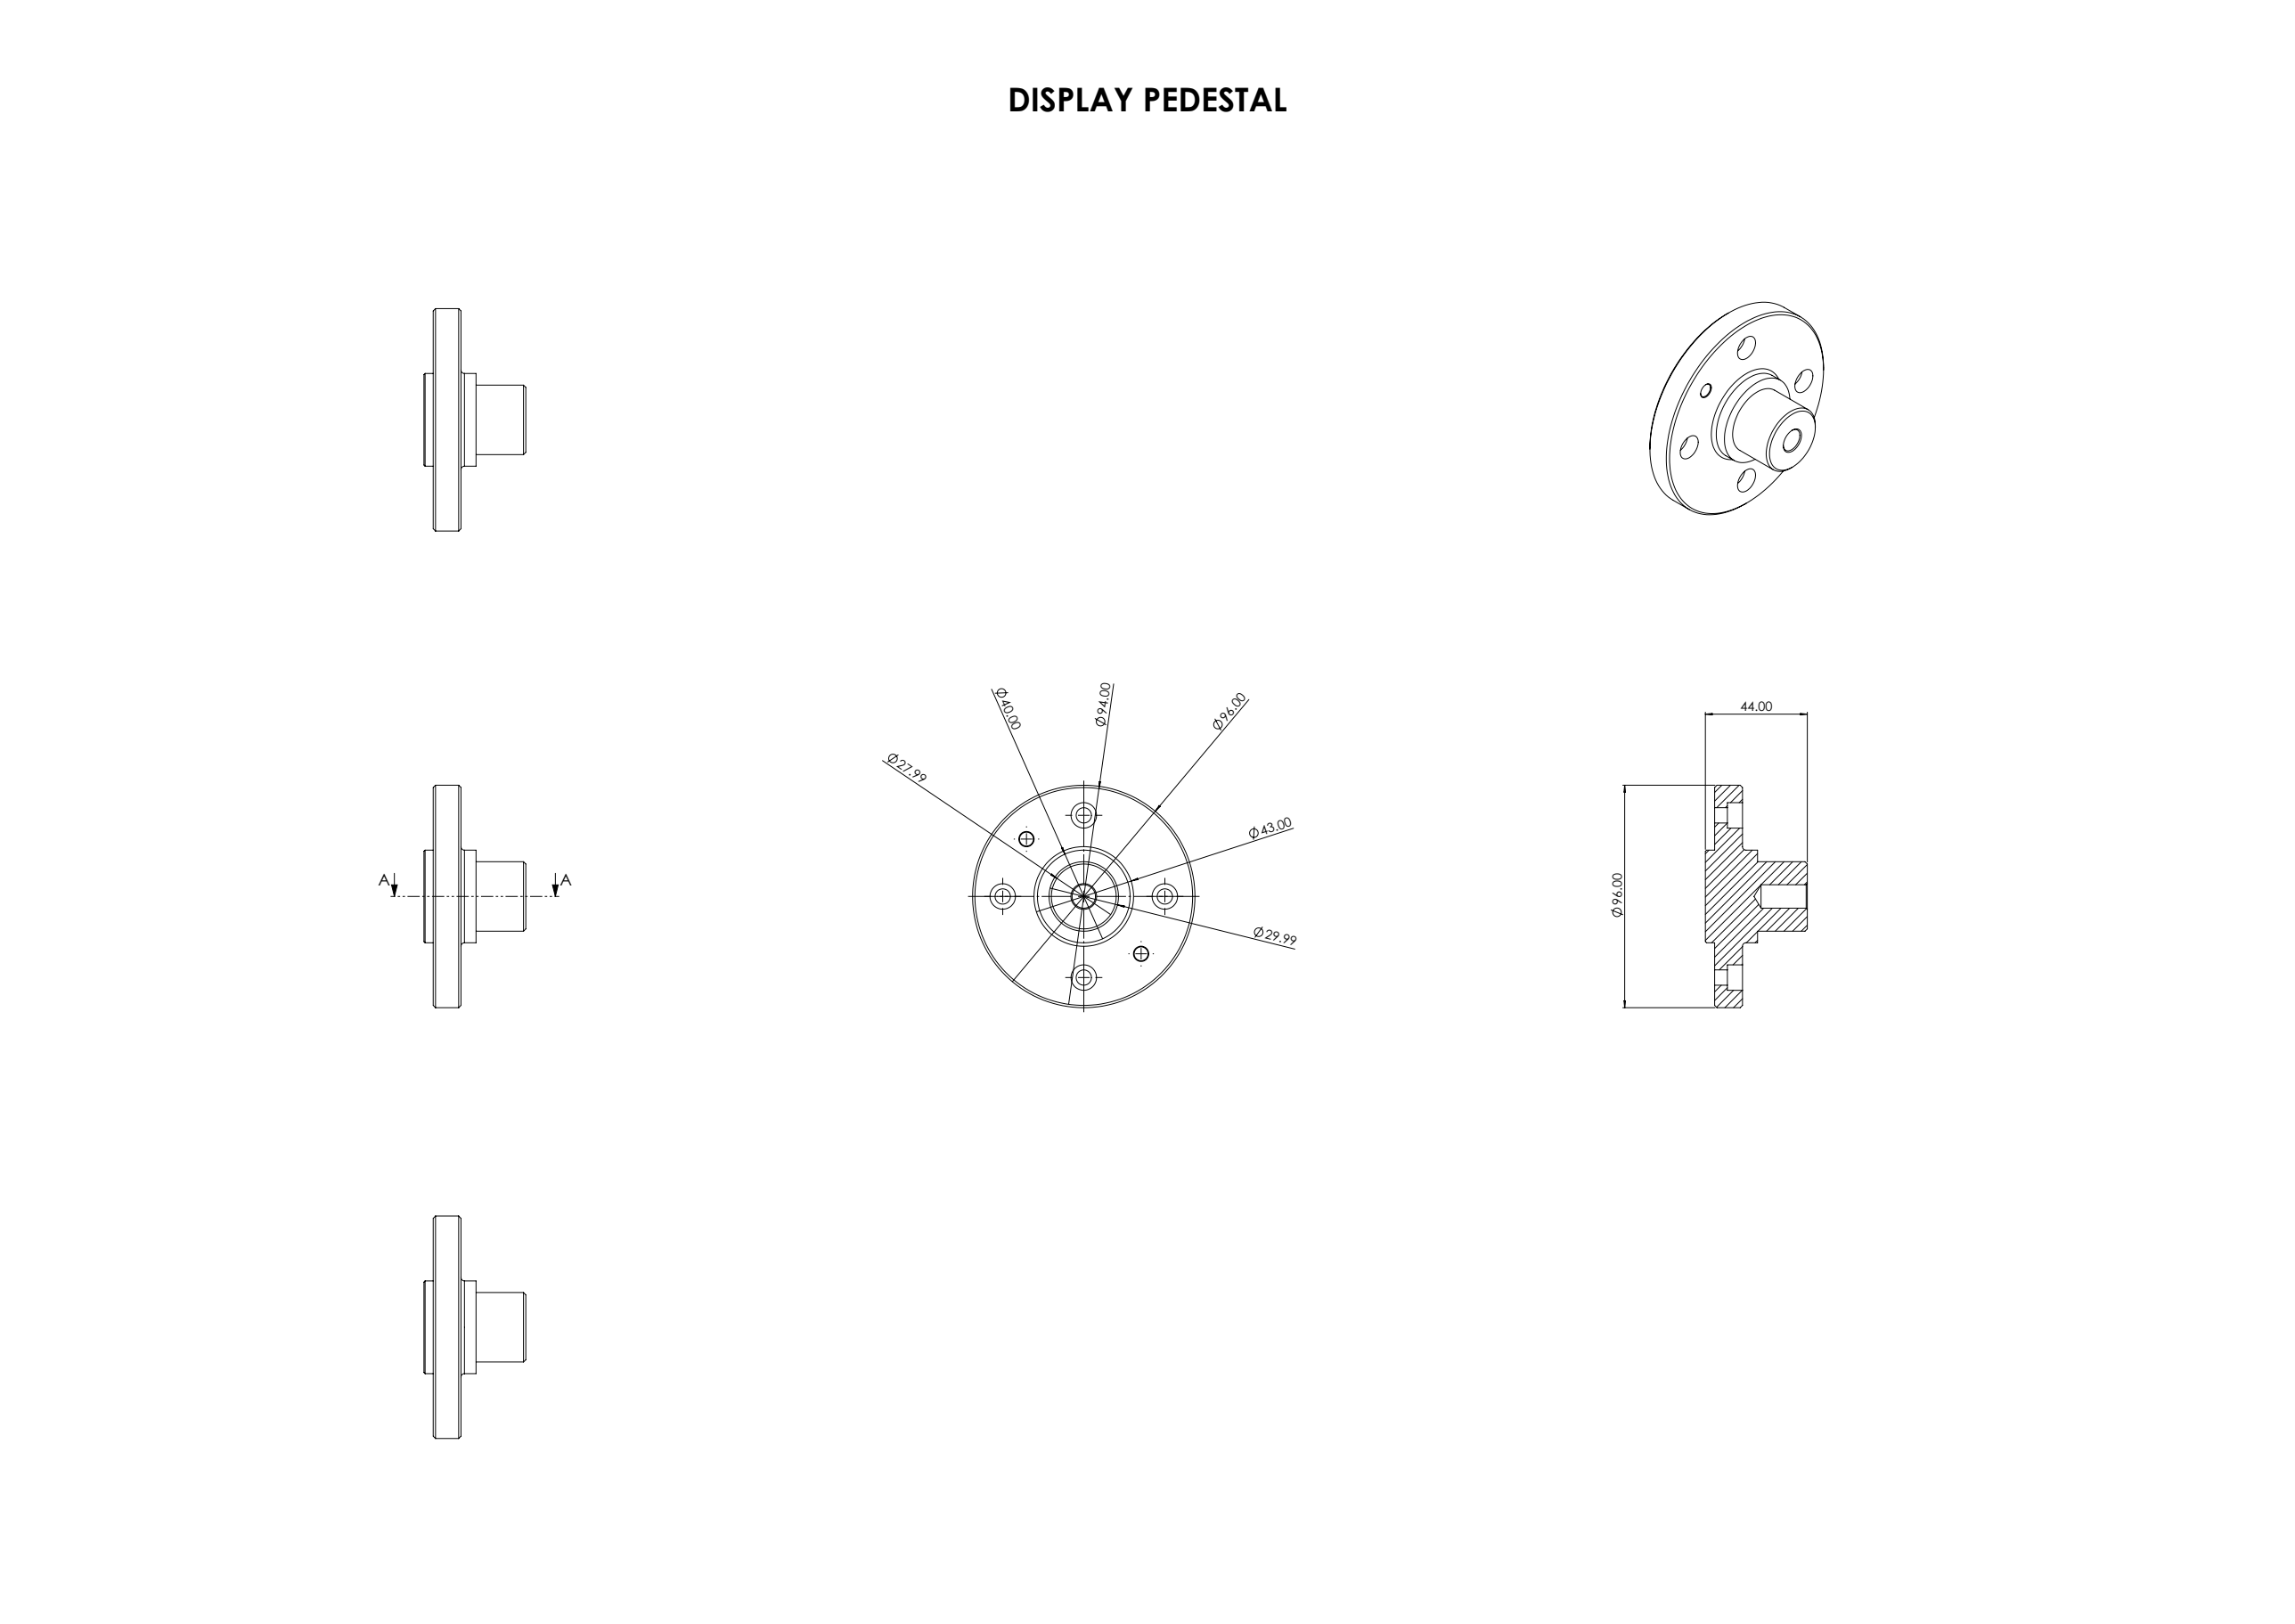
ISO-10303-21;
HEADER;
/* Generated by software containing ST-Developer
 * from STEP Tools, Inc. (www.steptools.com) 
 */

FILE_DESCRIPTION(
/* description */ (''),
/* implementation_level */ '2;1');

FILE_NAME(
/* name */ '03_Display_Pedestal.step',
/* time_stamp */ '2026-10-11T08:27:52-07:00',
/* author */ (''),
/* organization */ (''),
/* preprocessor_version */ 'ST-DEVELOPER v20.2',
/* originating_system */ 'Autodesk Translation Framework v15.15.0.0',
/* authorisation */ '');

FILE_SCHEMA (('AUTOMOTIVE_DESIGN { 1 0 10303 214 3 1 1 }'));
ENDSEC;

DATA;
#10=MECHANICAL_DESIGN_GEOMETRIC_PRESENTATION_REPRESENTATION('',(#921),#94301);
#893=SHAPE_REPRESENTATION_RELATIONSHIP('SRR','None',#94373,#907);
#907=ADVANCED_BREP_SHAPE_REPRESENTATION('',(#935),#94289);
#921=STYLED_ITEM('',(#94574),#935);
#935=MANIFOLD_SOLID_BREP('Body1',#51020);
#954=TOROIDAL_SURFACE('',#54190,21.5,1.5);
#969=FACE_BOUND('',#17694,.T.);
#970=FACE_BOUND('',#17695,.T.);
#971=FACE_BOUND('',#17696,.T.);
#972=FACE_BOUND('',#17697,.T.);
#973=FACE_BOUND('',#17698,.T.);
#974=FACE_BOUND('',#17699,.T.);
#975=FACE_BOUND('',#17700,.T.);
#976=FACE_BOUND('',#17710,.T.);
#977=FACE_BOUND('',#17713,.T.);
#978=FACE_BOUND('',#17716,.T.);
#979=FACE_BOUND('',#17719,.T.);
#980=FACE_BOUND('',#17729,.T.);
#981=FACE_BOUND('',#17730,.T.);
#982=FACE_BOUND('',#17731,.T.);
#983=FACE_BOUND('',#17732,.T.);
#984=FACE_BOUND('',#17733,.T.);
#985=FACE_BOUND('',#17734,.T.);
#986=FACE_BOUND('',#17735,.T.);
#987=FACE_BOUND('',#17740,.T.);
#988=FACE_BOUND('',#17744,.T.);
#1125=CYLINDRICAL_SURFACE('',#54154,3.);
#1126=CYLINDRICAL_SURFACE('',#54158,3.);
#1127=CYLINDRICAL_SURFACE('',#54160,3.3);
#1128=CYLINDRICAL_SURFACE('',#54163,3.3);
#1129=CYLINDRICAL_SURFACE('',#54166,3.3);
#1130=CYLINDRICAL_SURFACE('',#54169,3.3);
#1131=CYLINDRICAL_SURFACE('',#54172,5.5);
#1132=CYLINDRICAL_SURFACE('',#54175,5.5);
#1133=CYLINDRICAL_SURFACE('',#54178,5.5);
#1134=CYLINDRICAL_SURFACE('',#54181,5.5);
#1135=CYLINDRICAL_SURFACE('',#54186,5.05);
#1136=CYLINDRICAL_SURFACE('',#54194,20.);
#1137=CYLINDRICAL_SURFACE('',#54200,20.);
#1138=CYLINDRICAL_SURFACE('',#54206,48.);
#1139=CYLINDRICAL_SURFACE('',#54211,14.995);
#5334=LINE('',#80394,#9862);
#5335=LINE('',#80414,#9863);
#5336=LINE('',#80417,#9864);
#5337=LINE('',#80422,#9865);
#5338=LINE('',#80427,#9866);
#5339=LINE('',#80433,#9867);
#5340=LINE('',#80439,#9868);
#5341=LINE('',#80445,#9869);
#5342=LINE('',#80450,#9870);
#5343=LINE('',#80455,#9871);
#5344=LINE('',#80460,#9872);
#5345=LINE('',#80465,#9873);
#5346=LINE('',#80470,#9874);
#5347=LINE('',#80474,#9875);
#5348=LINE('',#80478,#9876);
#5349=LINE('',#80489,#9877);
#5350=LINE('',#80496,#9878);
#5351=LINE('',#80500,#9879);
#5352=LINE('',#80507,#9880);
#5353=LINE('',#80511,#9881);
#5354=LINE('',#80513,#9882);
#5355=LINE('',#80520,#9883);
#5356=LINE('',#80524,#9884);
#9862=VECTOR('',#64458,3.15);
#9863=VECTOR('',#64481,3.);
#9864=VECTOR('',#64484,3.15);
#9865=VECTOR('',#64491,3.);
#9866=VECTOR('',#64496,3.3);
#9867=VECTOR('',#64503,3.3);
#9868=VECTOR('',#64510,3.3);
#9869=VECTOR('',#64517,3.3);
#9870=VECTOR('',#64524,5.5);
#9871=VECTOR('',#64531,5.5);
#9872=VECTOR('',#64538,5.5);
#9873=VECTOR('',#64545,5.5);
#9874=VECTOR('',#64550,2.525);
#9875=VECTOR('',#64555,5.05);
#9876=VECTOR('',#64560,5.35);
#9877=VECTOR('',#64575,20.);
#9878=VECTOR('',#64584,19.75);
#9879=VECTOR('',#64589,20.);
#9880=VECTOR('',#64598,47.5);
#9881=VECTOR('',#64603,48.);
#9882=VECTOR('',#64606,47.5);
#9883=VECTOR('',#64615,14.995);
#9884=VECTOR('',#64620,14.495);
#12726=PLANE('',#54146);
#12727=PLANE('',#54174);
#12728=PLANE('',#54177);
#12729=PLANE('',#54180);
#12730=PLANE('',#54183);
#12731=PLANE('',#54196);
#12732=PLANE('',#54202);
#12733=PLANE('',#54209);
#12734=PLANE('',#54215);
#15000=FACE_OUTER_BOUND('',#17692,.T.);
#15001=FACE_OUTER_BOUND('',#17693,.T.);
#15002=FACE_OUTER_BOUND('',#17701,.T.);
#15003=FACE_OUTER_BOUND('',#17702,.T.);
#15004=FACE_OUTER_BOUND('',#17703,.T.);
#15005=FACE_OUTER_BOUND('',#17704,.T.);
#15006=FACE_OUTER_BOUND('',#17705,.T.);
#15007=FACE_OUTER_BOUND('',#17706,.T.);
#15008=FACE_OUTER_BOUND('',#17707,.T.);
#15009=FACE_OUTER_BOUND('',#17708,.T.);
#15010=FACE_OUTER_BOUND('',#17709,.T.);
#15011=FACE_OUTER_BOUND('',#17711,.T.);
#15012=FACE_OUTER_BOUND('',#17712,.T.);
#15013=FACE_OUTER_BOUND('',#17714,.T.);
#15014=FACE_OUTER_BOUND('',#17715,.T.);
#15015=FACE_OUTER_BOUND('',#17717,.T.);
#15016=FACE_OUTER_BOUND('',#17718,.T.);
#15017=FACE_OUTER_BOUND('',#17720,.T.);
#15018=FACE_OUTER_BOUND('',#17721,.T.);
#15019=FACE_OUTER_BOUND('',#17722,.T.);
#15020=FACE_OUTER_BOUND('',#17723,.T.);
#15021=FACE_OUTER_BOUND('',#17724,.T.);
#15022=FACE_OUTER_BOUND('',#17725,.T.);
#15023=FACE_OUTER_BOUND('',#17726,.T.);
#15024=FACE_OUTER_BOUND('',#17727,.T.);
#15025=FACE_OUTER_BOUND('',#17728,.T.);
#15026=FACE_OUTER_BOUND('',#17736,.T.);
#15027=FACE_OUTER_BOUND('',#17737,.T.);
#15028=FACE_OUTER_BOUND('',#17738,.T.);
#15029=FACE_OUTER_BOUND('',#17739,.T.);
#15030=FACE_OUTER_BOUND('',#17741,.T.);
#15031=FACE_OUTER_BOUND('',#17742,.T.);
#15032=FACE_OUTER_BOUND('',#17743,.T.);
#17692=EDGE_LOOP('',(#43353,#43354,#43355,#43356));
#17693=EDGE_LOOP('',(#43357));
#17694=EDGE_LOOP('',(#43358));
#17695=EDGE_LOOP('',(#43359));
#17696=EDGE_LOOP('',(#43360));
#17697=EDGE_LOOP('',(#43361));
#17698=EDGE_LOOP('',(#43362));
#17699=EDGE_LOOP('',(#43363));
#17700=EDGE_LOOP('',(#43364));
#17701=EDGE_LOOP('',(#43365,#43366,#43367,#43368));
#17702=EDGE_LOOP('',(#43369,#43370,#43371,#43372));
#17703=EDGE_LOOP('',(#43373,#43374,#43375,#43376));
#17704=EDGE_LOOP('',(#43377,#43378,#43379,#43380));
#17705=EDGE_LOOP('',(#43381,#43382,#43383,#43384));
#17706=EDGE_LOOP('',(#43385,#43386,#43387,#43388));
#17707=EDGE_LOOP('',(#43389,#43390,#43391,#43392));
#17708=EDGE_LOOP('',(#43393,#43394,#43395,#43396));
#17709=EDGE_LOOP('',(#43397));
#17710=EDGE_LOOP('',(#43398));
#17711=EDGE_LOOP('',(#43399,#43400,#43401,#43402));
#17712=EDGE_LOOP('',(#43403));
#17713=EDGE_LOOP('',(#43404));
#17714=EDGE_LOOP('',(#43405,#43406,#43407,#43408));
#17715=EDGE_LOOP('',(#43409));
#17716=EDGE_LOOP('',(#43410));
#17717=EDGE_LOOP('',(#43411,#43412,#43413,#43414));
#17718=EDGE_LOOP('',(#43415));
#17719=EDGE_LOOP('',(#43416));
#17720=EDGE_LOOP('',(#43417,#43418,#43419));
#17721=EDGE_LOOP('',(#43420,#43421,#43422,#43423));
#17722=EDGE_LOOP('',(#43424,#43425,#43426,#43427));
#17723=EDGE_LOOP('',(#43428,#43429,#43430,#43431,#43432));
#17724=EDGE_LOOP('',(#43433,#43434,#43435,#43436,#43437));
#17725=EDGE_LOOP('',(#43438));
#17726=EDGE_LOOP('',(#43439,#43440,#43441,#43442));
#17727=EDGE_LOOP('',(#43443,#43444,#43445,#43446));
#17728=EDGE_LOOP('',(#43447));
#17729=EDGE_LOOP('',(#43448));
#17730=EDGE_LOOP('',(#43449));
#17731=EDGE_LOOP('',(#43450));
#17732=EDGE_LOOP('',(#43451));
#17733=EDGE_LOOP('',(#43452));
#17734=EDGE_LOOP('',(#43453));
#17735=EDGE_LOOP('',(#43454));
#17736=EDGE_LOOP('',(#43455,#43456,#43457,#43458));
#17737=EDGE_LOOP('',(#43459,#43460,#43461,#43462));
#17738=EDGE_LOOP('',(#43463,#43464,#43465,#43466));
#17739=EDGE_LOOP('',(#43467));
#17740=EDGE_LOOP('',(#43468));
#17741=EDGE_LOOP('',(#43469,#43470,#43471,#43472));
#17742=EDGE_LOOP('',(#43473,#43474,#43475,#43476));
#17743=EDGE_LOOP('',(#43477));
#17744=EDGE_LOOP('',(#43478));
#19911=CIRCLE('',#54144,3.3);
#19912=CIRCLE('',#54145,3.);
#19913=CIRCLE('',#54147,47.);
#19914=CIRCLE('',#54148,3.3);
#19915=CIRCLE('',#54149,5.5);
#19916=CIRCLE('',#54150,5.5);
#19917=CIRCLE('',#54151,5.5);
#19918=CIRCLE('',#54152,5.5);
#19919=CIRCLE('',#54153,21.5);
#19920=CIRCLE('',#54155,3.);
#19921=CIRCLE('',#54157,3.);
#19922=CIRCLE('',#54159,3.);
#19923=CIRCLE('',#54161,3.3);
#19924=CIRCLE('',#54162,3.3);
#19925=CIRCLE('',#54164,3.3);
#19926=CIRCLE('',#54165,3.3);
#19927=CIRCLE('',#54167,3.3);
#19928=CIRCLE('',#54168,3.3);
#19929=CIRCLE('',#54170,3.3);
#19930=CIRCLE('',#54171,3.3);
#19931=CIRCLE('',#54173,5.5);
#19932=CIRCLE('',#54176,5.5);
#19933=CIRCLE('',#54179,5.5);
#19934=CIRCLE('',#54182,5.5);
#19935=CIRCLE('',#54185,5.05);
#19936=CIRCLE('',#54187,5.05);
#19937=CIRCLE('',#54189,5.55);
#19938=CIRCLE('',#54191,1.5);
#19939=CIRCLE('',#54192,20.);
#19940=CIRCLE('',#54193,20.);
#19941=CIRCLE('',#54195,20.);
#19942=CIRCLE('',#54197,19.5);
#19943=CIRCLE('',#54199,20.);
#19944=CIRCLE('',#54201,20.);
#19945=CIRCLE('',#54203,47.);
#19946=CIRCLE('',#54205,48.);
#19947=CIRCLE('',#54207,48.);
#19948=CIRCLE('',#54210,14.995);
#19949=CIRCLE('',#54212,14.995);
#19950=CIRCLE('',#54214,13.995);
#23800=VERTEX_POINT('',#80391);
#23801=VERTEX_POINT('',#80393);
#23802=VERTEX_POINT('',#80397);
#23803=VERTEX_POINT('',#80399);
#23804=VERTEX_POINT('',#80401);
#23805=VERTEX_POINT('',#80403);
#23806=VERTEX_POINT('',#80405);
#23807=VERTEX_POINT('',#80407);
#23808=VERTEX_POINT('',#80409);
#23809=VERTEX_POINT('',#80412);
#23810=VERTEX_POINT('',#80416);
#23811=VERTEX_POINT('',#80420);
#23812=VERTEX_POINT('',#80424);
#23813=VERTEX_POINT('',#80426);
#23814=VERTEX_POINT('',#80430);
#23815=VERTEX_POINT('',#80432);
#23816=VERTEX_POINT('',#80436);
#23817=VERTEX_POINT('',#80438);
#23818=VERTEX_POINT('',#80442);
#23819=VERTEX_POINT('',#80444);
#23820=VERTEX_POINT('',#80448);
#23821=VERTEX_POINT('',#80453);
#23822=VERTEX_POINT('',#80458);
#23823=VERTEX_POINT('',#80463);
#23824=VERTEX_POINT('',#80468);
#23825=VERTEX_POINT('',#80469);
#23826=VERTEX_POINT('',#80473);
#23827=VERTEX_POINT('',#80477);
#23828=VERTEX_POINT('',#80481);
#23829=VERTEX_POINT('',#80483);
#23830=VERTEX_POINT('',#80487);
#23831=VERTEX_POINT('',#80491);
#23832=VERTEX_POINT('',#80494);
#23833=VERTEX_POINT('',#80498);
#23834=VERTEX_POINT('',#80502);
#23835=VERTEX_POINT('',#80505);
#23836=VERTEX_POINT('',#80509);
#23837=VERTEX_POINT('',#80515);
#23838=VERTEX_POINT('',#80518);
#23839=VERTEX_POINT('',#80522);
#30538=EDGE_CURVE('',#23800,#23800,#19911,.T.);
#30539=EDGE_CURVE('',#23800,#23801,#5334,.T.);
#30540=EDGE_CURVE('',#23801,#23801,#19912,.T.);
#30541=EDGE_CURVE('',#23802,#23802,#19913,.T.);
#30542=EDGE_CURVE('',#23803,#23803,#19914,.T.);
#30543=EDGE_CURVE('',#23804,#23804,#19915,.T.);
#30544=EDGE_CURVE('',#23805,#23805,#19916,.T.);
#30545=EDGE_CURVE('',#23806,#23806,#19917,.T.);
#30546=EDGE_CURVE('',#23807,#23807,#19918,.T.);
#30547=EDGE_CURVE('',#23808,#23808,#19919,.T.);
#30548=EDGE_CURVE('',#23809,#23809,#19920,.T.);
#30549=EDGE_CURVE('',#23809,#23801,#5335,.T.);
#30550=EDGE_CURVE('',#23803,#23810,#5336,.T.);
#30551=EDGE_CURVE('',#23810,#23810,#19921,.T.);
#30552=EDGE_CURVE('',#23811,#23811,#19922,.T.);
#30553=EDGE_CURVE('',#23811,#23810,#5337,.T.);
#30554=EDGE_CURVE('',#23812,#23812,#19923,.T.);
#30555=EDGE_CURVE('',#23812,#23813,#5338,.T.);
#30556=EDGE_CURVE('',#23813,#23813,#19924,.T.);
#30557=EDGE_CURVE('',#23814,#23814,#19925,.T.);
#30558=EDGE_CURVE('',#23814,#23815,#5339,.T.);
#30559=EDGE_CURVE('',#23815,#23815,#19926,.T.);
#30560=EDGE_CURVE('',#23816,#23816,#19927,.T.);
#30561=EDGE_CURVE('',#23816,#23817,#5340,.T.);
#30562=EDGE_CURVE('',#23817,#23817,#19928,.T.);
#30563=EDGE_CURVE('',#23818,#23818,#19929,.T.);
#30564=EDGE_CURVE('',#23818,#23819,#5341,.T.);
#30565=EDGE_CURVE('',#23819,#23819,#19930,.T.);
#30566=EDGE_CURVE('',#23820,#23820,#19931,.T.);
#30567=EDGE_CURVE('',#23820,#23804,#5342,.T.);
#30568=EDGE_CURVE('',#23821,#23821,#19932,.T.);
#30569=EDGE_CURVE('',#23821,#23805,#5343,.T.);
#30570=EDGE_CURVE('',#23822,#23822,#19933,.T.);
#30571=EDGE_CURVE('',#23822,#23806,#5344,.T.);
#30572=EDGE_CURVE('',#23823,#23823,#19934,.T.);
#30573=EDGE_CURVE('',#23823,#23807,#5345,.T.);
#30574=EDGE_CURVE('',#23824,#23825,#5346,.T.);
#30575=EDGE_CURVE('',#23825,#23825,#19935,.T.);
#30576=EDGE_CURVE('',#23825,#23826,#5347,.T.);
#30577=EDGE_CURVE('',#23826,#23826,#19936,.T.);
#30578=EDGE_CURVE('',#23826,#23827,#5348,.T.);
#30579=EDGE_CURVE('',#23827,#23827,#19937,.T.);
#30580=EDGE_CURVE('',#23808,#23828,#19938,.T.);
#30581=EDGE_CURVE('',#23828,#23829,#19939,.T.);
#30582=EDGE_CURVE('',#23829,#23828,#19940,.T.);
#30583=EDGE_CURVE('',#23830,#23830,#19941,.T.);
#30584=EDGE_CURVE('',#23830,#23829,#5349,.T.);
#30585=EDGE_CURVE('',#23831,#23831,#19942,.T.);
#30586=EDGE_CURVE('',#23832,#23832,#19943,.T.);
#30587=EDGE_CURVE('',#23832,#23831,#5350,.T.);
#30588=EDGE_CURVE('',#23833,#23833,#19944,.T.);
#30589=EDGE_CURVE('',#23833,#23832,#5351,.T.);
#30590=EDGE_CURVE('',#23834,#23834,#19945,.T.);
#30591=EDGE_CURVE('',#23835,#23835,#19946,.T.);
#30592=EDGE_CURVE('',#23835,#23834,#5352,.T.);
#30593=EDGE_CURVE('',#23836,#23836,#19947,.T.);
#30594=EDGE_CURVE('',#23836,#23835,#5353,.T.);
#30595=EDGE_CURVE('',#23802,#23836,#5354,.T.);
#30596=EDGE_CURVE('',#23837,#23837,#19948,.T.);
#30597=EDGE_CURVE('',#23838,#23838,#19949,.T.);
#30598=EDGE_CURVE('',#23838,#23837,#5355,.T.);
#30599=EDGE_CURVE('',#23839,#23839,#19950,.T.);
#30600=EDGE_CURVE('',#23839,#23838,#5356,.T.);
#43353=ORIENTED_EDGE('',*,*,#30538,.T.);
#43354=ORIENTED_EDGE('',*,*,#30539,.T.);
#43355=ORIENTED_EDGE('',*,*,#30540,.T.);
#43356=ORIENTED_EDGE('',*,*,#30539,.F.);
#43357=ORIENTED_EDGE('',*,*,#30541,.T.);
#43358=ORIENTED_EDGE('',*,*,#30542,.F.);
#43359=ORIENTED_EDGE('',*,*,#30543,.T.);
#43360=ORIENTED_EDGE('',*,*,#30544,.T.);
#43361=ORIENTED_EDGE('',*,*,#30545,.T.);
#43362=ORIENTED_EDGE('',*,*,#30546,.T.);
#43363=ORIENTED_EDGE('',*,*,#30547,.F.);
#43364=ORIENTED_EDGE('',*,*,#30538,.F.);
#43365=ORIENTED_EDGE('',*,*,#30548,.F.);
#43366=ORIENTED_EDGE('',*,*,#30549,.T.);
#43367=ORIENTED_EDGE('',*,*,#30540,.F.);
#43368=ORIENTED_EDGE('',*,*,#30549,.F.);
#43369=ORIENTED_EDGE('',*,*,#30542,.T.);
#43370=ORIENTED_EDGE('',*,*,#30550,.T.);
#43371=ORIENTED_EDGE('',*,*,#30551,.T.);
#43372=ORIENTED_EDGE('',*,*,#30550,.F.);
#43373=ORIENTED_EDGE('',*,*,#30552,.F.);
#43374=ORIENTED_EDGE('',*,*,#30553,.T.);
#43375=ORIENTED_EDGE('',*,*,#30551,.F.);
#43376=ORIENTED_EDGE('',*,*,#30553,.F.);
#43377=ORIENTED_EDGE('',*,*,#30554,.F.);
#43378=ORIENTED_EDGE('',*,*,#30555,.T.);
#43379=ORIENTED_EDGE('',*,*,#30556,.F.);
#43380=ORIENTED_EDGE('',*,*,#30555,.F.);
#43381=ORIENTED_EDGE('',*,*,#30557,.F.);
#43382=ORIENTED_EDGE('',*,*,#30558,.T.);
#43383=ORIENTED_EDGE('',*,*,#30559,.F.);
#43384=ORIENTED_EDGE('',*,*,#30558,.F.);
#43385=ORIENTED_EDGE('',*,*,#30560,.F.);
#43386=ORIENTED_EDGE('',*,*,#30561,.T.);
#43387=ORIENTED_EDGE('',*,*,#30562,.F.);
#43388=ORIENTED_EDGE('',*,*,#30561,.F.);
#43389=ORIENTED_EDGE('',*,*,#30563,.F.);
#43390=ORIENTED_EDGE('',*,*,#30564,.T.);
#43391=ORIENTED_EDGE('',*,*,#30565,.F.);
#43392=ORIENTED_EDGE('',*,*,#30564,.F.);
#43393=ORIENTED_EDGE('',*,*,#30566,.F.);
#43394=ORIENTED_EDGE('',*,*,#30567,.T.);
#43395=ORIENTED_EDGE('',*,*,#30543,.F.);
#43396=ORIENTED_EDGE('',*,*,#30567,.F.);
#43397=ORIENTED_EDGE('',*,*,#30566,.T.);
#43398=ORIENTED_EDGE('',*,*,#30562,.T.);
#43399=ORIENTED_EDGE('',*,*,#30568,.F.);
#43400=ORIENTED_EDGE('',*,*,#30569,.T.);
#43401=ORIENTED_EDGE('',*,*,#30544,.F.);
#43402=ORIENTED_EDGE('',*,*,#30569,.F.);
#43403=ORIENTED_EDGE('',*,*,#30568,.T.);
#43404=ORIENTED_EDGE('',*,*,#30559,.T.);
#43405=ORIENTED_EDGE('',*,*,#30570,.F.);
#43406=ORIENTED_EDGE('',*,*,#30571,.T.);
#43407=ORIENTED_EDGE('',*,*,#30545,.F.);
#43408=ORIENTED_EDGE('',*,*,#30571,.F.);
#43409=ORIENTED_EDGE('',*,*,#30570,.T.);
#43410=ORIENTED_EDGE('',*,*,#30556,.T.);
#43411=ORIENTED_EDGE('',*,*,#30572,.F.);
#43412=ORIENTED_EDGE('',*,*,#30573,.T.);
#43413=ORIENTED_EDGE('',*,*,#30546,.F.);
#43414=ORIENTED_EDGE('',*,*,#30573,.F.);
#43415=ORIENTED_EDGE('',*,*,#30572,.T.);
#43416=ORIENTED_EDGE('',*,*,#30565,.T.);
#43417=ORIENTED_EDGE('',*,*,#30574,.T.);
#43418=ORIENTED_EDGE('',*,*,#30575,.T.);
#43419=ORIENTED_EDGE('',*,*,#30574,.F.);
#43420=ORIENTED_EDGE('',*,*,#30575,.F.);
#43421=ORIENTED_EDGE('',*,*,#30576,.T.);
#43422=ORIENTED_EDGE('',*,*,#30577,.T.);
#43423=ORIENTED_EDGE('',*,*,#30576,.F.);
#43424=ORIENTED_EDGE('',*,*,#30577,.F.);
#43425=ORIENTED_EDGE('',*,*,#30578,.T.);
#43426=ORIENTED_EDGE('',*,*,#30579,.F.);
#43427=ORIENTED_EDGE('',*,*,#30578,.F.);
#43428=ORIENTED_EDGE('',*,*,#30547,.T.);
#43429=ORIENTED_EDGE('',*,*,#30580,.T.);
#43430=ORIENTED_EDGE('',*,*,#30581,.T.);
#43431=ORIENTED_EDGE('',*,*,#30582,.T.);
#43432=ORIENTED_EDGE('',*,*,#30580,.F.);
#43433=ORIENTED_EDGE('',*,*,#30583,.F.);
#43434=ORIENTED_EDGE('',*,*,#30584,.T.);
#43435=ORIENTED_EDGE('',*,*,#30581,.F.);
#43436=ORIENTED_EDGE('',*,*,#30582,.F.);
#43437=ORIENTED_EDGE('',*,*,#30584,.F.);
#43438=ORIENTED_EDGE('',*,*,#30585,.F.);
#43439=ORIENTED_EDGE('',*,*,#30586,.F.);
#43440=ORIENTED_EDGE('',*,*,#30587,.T.);
#43441=ORIENTED_EDGE('',*,*,#30585,.T.);
#43442=ORIENTED_EDGE('',*,*,#30587,.F.);
#43443=ORIENTED_EDGE('',*,*,#30588,.F.);
#43444=ORIENTED_EDGE('',*,*,#30589,.T.);
#43445=ORIENTED_EDGE('',*,*,#30586,.T.);
#43446=ORIENTED_EDGE('',*,*,#30589,.F.);
#43447=ORIENTED_EDGE('',*,*,#30590,.F.);
#43448=ORIENTED_EDGE('',*,*,#30588,.T.);
#43449=ORIENTED_EDGE('',*,*,#30548,.T.);
#43450=ORIENTED_EDGE('',*,*,#30563,.T.);
#43451=ORIENTED_EDGE('',*,*,#30560,.T.);
#43452=ORIENTED_EDGE('',*,*,#30557,.T.);
#43453=ORIENTED_EDGE('',*,*,#30554,.T.);
#43454=ORIENTED_EDGE('',*,*,#30552,.T.);
#43455=ORIENTED_EDGE('',*,*,#30591,.F.);
#43456=ORIENTED_EDGE('',*,*,#30592,.T.);
#43457=ORIENTED_EDGE('',*,*,#30590,.T.);
#43458=ORIENTED_EDGE('',*,*,#30592,.F.);
#43459=ORIENTED_EDGE('',*,*,#30593,.F.);
#43460=ORIENTED_EDGE('',*,*,#30594,.T.);
#43461=ORIENTED_EDGE('',*,*,#30591,.T.);
#43462=ORIENTED_EDGE('',*,*,#30594,.F.);
#43463=ORIENTED_EDGE('',*,*,#30541,.F.);
#43464=ORIENTED_EDGE('',*,*,#30595,.T.);
#43465=ORIENTED_EDGE('',*,*,#30593,.T.);
#43466=ORIENTED_EDGE('',*,*,#30595,.F.);
#43467=ORIENTED_EDGE('',*,*,#30583,.T.);
#43468=ORIENTED_EDGE('',*,*,#30596,.F.);
#43469=ORIENTED_EDGE('',*,*,#30597,.F.);
#43470=ORIENTED_EDGE('',*,*,#30598,.T.);
#43471=ORIENTED_EDGE('',*,*,#30596,.T.);
#43472=ORIENTED_EDGE('',*,*,#30598,.F.);
#43473=ORIENTED_EDGE('',*,*,#30599,.F.);
#43474=ORIENTED_EDGE('',*,*,#30600,.T.);
#43475=ORIENTED_EDGE('',*,*,#30597,.T.);
#43476=ORIENTED_EDGE('',*,*,#30600,.F.);
#43477=ORIENTED_EDGE('',*,*,#30599,.T.);
#43478=ORIENTED_EDGE('',*,*,#30579,.T.);
#48268=CONICAL_SURFACE('',#54143,3.15,0.785398163397444);
#48269=CONICAL_SURFACE('',#54156,3.15,0.785398163397444);
#48270=CONICAL_SURFACE('',#54184,2.525,1.02974425867665);
#48271=CONICAL_SURFACE('',#54188,5.35,0.785398163397451);
#48272=CONICAL_SURFACE('',#54198,19.75,0.785398163397448);
#48273=CONICAL_SURFACE('',#54204,47.5,0.785398163397447);
#48274=CONICAL_SURFACE('',#54208,47.5,0.785398163397447);
#48275=CONICAL_SURFACE('',#54213,14.495,0.785398163397447);
#50087=ADVANCED_FACE('',(#15000),#48268,.F.);
#50088=ADVANCED_FACE('',(#15001,#969,#970,#971,#972,#973,#974,#975),#12726,
 .T.);
#50089=ADVANCED_FACE('',(#15002),#1125,.F.);
#50090=ADVANCED_FACE('',(#15003),#48269,.F.);
#50091=ADVANCED_FACE('',(#15004),#1126,.F.);
#50092=ADVANCED_FACE('',(#15005),#1127,.F.);
#50093=ADVANCED_FACE('',(#15006),#1128,.F.);
#50094=ADVANCED_FACE('',(#15007),#1129,.F.);
#50095=ADVANCED_FACE('',(#15008),#1130,.F.);
#50096=ADVANCED_FACE('',(#15009),#1131,.F.);
#50097=ADVANCED_FACE('',(#15010,#976),#12727,.T.);
#50098=ADVANCED_FACE('',(#15011),#1132,.F.);
#50099=ADVANCED_FACE('',(#15012,#977),#12728,.T.);
#50100=ADVANCED_FACE('',(#15013),#1133,.F.);
#50101=ADVANCED_FACE('',(#15014,#978),#12729,.T.);
#50102=ADVANCED_FACE('',(#15015),#1134,.F.);
#50103=ADVANCED_FACE('',(#15016,#979),#12730,.T.);
#50104=ADVANCED_FACE('',(#15017),#48270,.F.);
#50105=ADVANCED_FACE('',(#15018),#1135,.F.);
#50106=ADVANCED_FACE('',(#15019),#48271,.F.);
#50107=ADVANCED_FACE('',(#15020),#954,.F.);
#50108=ADVANCED_FACE('',(#15021),#1136,.T.);
#50109=ADVANCED_FACE('',(#15022),#12731,.T.);
#50110=ADVANCED_FACE('',(#15023),#48272,.T.);
#50111=ADVANCED_FACE('',(#15024),#1137,.T.);
#50112=ADVANCED_FACE('',(#15025,#980,#981,#982,#983,#984,#985,#986),#12732,
 .T.);
#50113=ADVANCED_FACE('',(#15026),#48273,.T.);
#50114=ADVANCED_FACE('',(#15027),#1138,.T.);
#50115=ADVANCED_FACE('',(#15028),#48274,.T.);
#50116=ADVANCED_FACE('',(#15029,#987),#12733,.T.);
#50117=ADVANCED_FACE('',(#15030),#1139,.T.);
#50118=ADVANCED_FACE('',(#15031),#48275,.T.);
#50119=ADVANCED_FACE('',(#15032,#988),#12734,.T.);
#51020=CLOSED_SHELL('',(#50087,#50088,#50089,#50090,#50091,#50092,#50093,
#50094,#50095,#50096,#50097,#50098,#50099,#50100,#50101,#50102,#50103,#50104,
#50105,#50106,#50107,#50108,#50109,#50110,#50111,#50112,#50113,#50114,#50115,
#50116,#50117,#50118,#50119));
#54142=AXIS2_PLACEMENT_3D('',#80389,#64452,#64453);
#54143=AXIS2_PLACEMENT_3D('',#80390,#64454,#64455);
#54144=AXIS2_PLACEMENT_3D('',#80392,#64456,#64457);
#54145=AXIS2_PLACEMENT_3D('',#80395,#64459,#64460);
#54146=AXIS2_PLACEMENT_3D('',#80396,#64461,#64462);
#54147=AXIS2_PLACEMENT_3D('',#80398,#64463,#64464);
#54148=AXIS2_PLACEMENT_3D('',#80400,#64465,#64466);
#54149=AXIS2_PLACEMENT_3D('',#80402,#64467,#64468);
#54150=AXIS2_PLACEMENT_3D('',#80404,#64469,#64470);
#54151=AXIS2_PLACEMENT_3D('',#80406,#64471,#64472);
#54152=AXIS2_PLACEMENT_3D('',#80408,#64473,#64474);
#54153=AXIS2_PLACEMENT_3D('',#80410,#64475,#64476);
#54154=AXIS2_PLACEMENT_3D('',#80411,#64477,#64478);
#54155=AXIS2_PLACEMENT_3D('',#80413,#64479,#64480);
#54156=AXIS2_PLACEMENT_3D('',#80415,#64482,#64483);
#54157=AXIS2_PLACEMENT_3D('',#80418,#64485,#64486);
#54158=AXIS2_PLACEMENT_3D('',#80419,#64487,#64488);
#54159=AXIS2_PLACEMENT_3D('',#80421,#64489,#64490);
#54160=AXIS2_PLACEMENT_3D('',#80423,#64492,#64493);
#54161=AXIS2_PLACEMENT_3D('',#80425,#64494,#64495);
#54162=AXIS2_PLACEMENT_3D('',#80428,#64497,#64498);
#54163=AXIS2_PLACEMENT_3D('',#80429,#64499,#64500);
#54164=AXIS2_PLACEMENT_3D('',#80431,#64501,#64502);
#54165=AXIS2_PLACEMENT_3D('',#80434,#64504,#64505);
#54166=AXIS2_PLACEMENT_3D('',#80435,#64506,#64507);
#54167=AXIS2_PLACEMENT_3D('',#80437,#64508,#64509);
#54168=AXIS2_PLACEMENT_3D('',#80440,#64511,#64512);
#54169=AXIS2_PLACEMENT_3D('',#80441,#64513,#64514);
#54170=AXIS2_PLACEMENT_3D('',#80443,#64515,#64516);
#54171=AXIS2_PLACEMENT_3D('',#80446,#64518,#64519);
#54172=AXIS2_PLACEMENT_3D('',#80447,#64520,#64521);
#54173=AXIS2_PLACEMENT_3D('',#80449,#64522,#64523);
#54174=AXIS2_PLACEMENT_3D('',#80451,#64525,#64526);
#54175=AXIS2_PLACEMENT_3D('',#80452,#64527,#64528);
#54176=AXIS2_PLACEMENT_3D('',#80454,#64529,#64530);
#54177=AXIS2_PLACEMENT_3D('',#80456,#64532,#64533);
#54178=AXIS2_PLACEMENT_3D('',#80457,#64534,#64535);
#54179=AXIS2_PLACEMENT_3D('',#80459,#64536,#64537);
#54180=AXIS2_PLACEMENT_3D('',#80461,#64539,#64540);
#54181=AXIS2_PLACEMENT_3D('',#80462,#64541,#64542);
#54182=AXIS2_PLACEMENT_3D('',#80464,#64543,#64544);
#54183=AXIS2_PLACEMENT_3D('',#80466,#64546,#64547);
#54184=AXIS2_PLACEMENT_3D('',#80467,#64548,#64549);
#54185=AXIS2_PLACEMENT_3D('',#80471,#64551,#64552);
#54186=AXIS2_PLACEMENT_3D('',#80472,#64553,#64554);
#54187=AXIS2_PLACEMENT_3D('',#80475,#64556,#64557);
#54188=AXIS2_PLACEMENT_3D('',#80476,#64558,#64559);
#54189=AXIS2_PLACEMENT_3D('',#80479,#64561,#64562);
#54190=AXIS2_PLACEMENT_3D('',#80480,#64563,#64564);
#54191=AXIS2_PLACEMENT_3D('',#80482,#64565,#64566);
#54192=AXIS2_PLACEMENT_3D('',#80484,#64567,#64568);
#54193=AXIS2_PLACEMENT_3D('',#80485,#64569,#64570);
#54194=AXIS2_PLACEMENT_3D('',#80486,#64571,#64572);
#54195=AXIS2_PLACEMENT_3D('',#80488,#64573,#64574);
#54196=AXIS2_PLACEMENT_3D('',#80490,#64576,#64577);
#54197=AXIS2_PLACEMENT_3D('',#80492,#64578,#64579);
#54198=AXIS2_PLACEMENT_3D('',#80493,#64580,#64581);
#54199=AXIS2_PLACEMENT_3D('',#80495,#64582,#64583);
#54200=AXIS2_PLACEMENT_3D('',#80497,#64585,#64586);
#54201=AXIS2_PLACEMENT_3D('',#80499,#64587,#64588);
#54202=AXIS2_PLACEMENT_3D('',#80501,#64590,#64591);
#54203=AXIS2_PLACEMENT_3D('',#80503,#64592,#64593);
#54204=AXIS2_PLACEMENT_3D('',#80504,#64594,#64595);
#54205=AXIS2_PLACEMENT_3D('',#80506,#64596,#64597);
#54206=AXIS2_PLACEMENT_3D('',#80508,#64599,#64600);
#54207=AXIS2_PLACEMENT_3D('',#80510,#64601,#64602);
#54208=AXIS2_PLACEMENT_3D('',#80512,#64604,#64605);
#54209=AXIS2_PLACEMENT_3D('',#80514,#64607,#64608);
#54210=AXIS2_PLACEMENT_3D('',#80516,#64609,#64610);
#54211=AXIS2_PLACEMENT_3D('',#80517,#64611,#64612);
#54212=AXIS2_PLACEMENT_3D('',#80519,#64613,#64614);
#54213=AXIS2_PLACEMENT_3D('',#80521,#64616,#64617);
#54214=AXIS2_PLACEMENT_3D('',#80523,#64618,#64619);
#54215=AXIS2_PLACEMENT_3D('',#80525,#64621,#64622);
#64452=DIRECTION('axis',(0.,0.,1.));
#64453=DIRECTION('refdir',(1.,0.,0.));
#64454=DIRECTION('center_axis',(1.,0.,0.));
#64455=DIRECTION('ref_axis',(0.,0.,-1.));
#64456=DIRECTION('center_axis',(1.,0.,0.));
#64457=DIRECTION('ref_axis',(0.,0.,-1.));
#64458=DIRECTION('',(-0.70710678118655,8.6595605623549E-17,-0.707106781186545));
#64459=DIRECTION('center_axis',(-1.,0.,0.));
#64460=DIRECTION('ref_axis',(0.,0.,-1.));
#64461=DIRECTION('center_axis',(1.,0.,0.));
#64462=DIRECTION('ref_axis',(0.,0.,-1.));
#64463=DIRECTION('center_axis',(1.,0.,0.));
#64464=DIRECTION('ref_axis',(0.,0.,-1.));
#64465=DIRECTION('center_axis',(1.,0.,0.));
#64466=DIRECTION('ref_axis',(0.,0.,-1.));
#64467=DIRECTION('center_axis',(-1.,0.,0.));
#64468=DIRECTION('ref_axis',(0.,0.,-1.));
#64469=DIRECTION('center_axis',(-1.,0.,0.));
#64470=DIRECTION('ref_axis',(0.,0.,-1.));
#64471=DIRECTION('center_axis',(-1.,0.,0.));
#64472=DIRECTION('ref_axis',(0.,0.,-1.));
#64473=DIRECTION('center_axis',(-1.,0.,0.));
#64474=DIRECTION('ref_axis',(0.,0.,-1.));
#64475=DIRECTION('center_axis',(1.,0.,0.));
#64476=DIRECTION('ref_axis',(0.,-1.,1.83697019872103E-16));
#64477=DIRECTION('center_axis',(1.,0.,0.));
#64478=DIRECTION('ref_axis',(0.,0.,-1.));
#64479=DIRECTION('center_axis',(1.,0.,0.));
#64480=DIRECTION('ref_axis',(0.,0.,-1.));
#64481=DIRECTION('',(1.,0.,0.));
#64482=DIRECTION('center_axis',(1.,0.,0.));
#64483=DIRECTION('ref_axis',(0.,0.,-1.));
#64484=DIRECTION('',(-0.70710678118655,8.6595605623549E-17,-0.707106781186545));
#64485=DIRECTION('center_axis',(-1.,0.,0.));
#64486=DIRECTION('ref_axis',(0.,0.,-1.));
#64487=DIRECTION('center_axis',(1.,0.,0.));
#64488=DIRECTION('ref_axis',(0.,0.,-1.));
#64489=DIRECTION('center_axis',(1.,0.,0.));
#64490=DIRECTION('ref_axis',(0.,0.,-1.));
#64491=DIRECTION('',(1.,0.,0.));
#64492=DIRECTION('center_axis',(1.,0.,0.));
#64493=DIRECTION('ref_axis',(0.,0.,-1.));
#64494=DIRECTION('center_axis',(1.,0.,0.));
#64495=DIRECTION('ref_axis',(0.,0.,-1.));
#64496=DIRECTION('',(1.,0.,0.));
#64497=DIRECTION('center_axis',(-1.,0.,0.));
#64498=DIRECTION('ref_axis',(0.,0.,-1.));
#64499=DIRECTION('center_axis',(1.,0.,0.));
#64500=DIRECTION('ref_axis',(0.,0.,-1.));
#64501=DIRECTION('center_axis',(1.,0.,0.));
#64502=DIRECTION('ref_axis',(0.,0.,-1.));
#64503=DIRECTION('',(1.,0.,0.));
#64504=DIRECTION('center_axis',(-1.,0.,0.));
#64505=DIRECTION('ref_axis',(0.,0.,-1.));
#64506=DIRECTION('center_axis',(1.,0.,0.));
#64507=DIRECTION('ref_axis',(0.,0.,-1.));
#64508=DIRECTION('center_axis',(1.,0.,0.));
#64509=DIRECTION('ref_axis',(0.,0.,-1.));
#64510=DIRECTION('',(1.,0.,0.));
#64511=DIRECTION('center_axis',(-1.,0.,0.));
#64512=DIRECTION('ref_axis',(0.,0.,-1.));
#64513=DIRECTION('center_axis',(1.,0.,0.));
#64514=DIRECTION('ref_axis',(0.,0.,-1.));
#64515=DIRECTION('center_axis',(1.,0.,0.));
#64516=DIRECTION('ref_axis',(0.,0.,-1.));
#64517=DIRECTION('',(1.,0.,0.));
#64518=DIRECTION('center_axis',(-1.,0.,0.));
#64519=DIRECTION('ref_axis',(0.,0.,-1.));
#64520=DIRECTION('center_axis',(1.,0.,0.));
#64521=DIRECTION('ref_axis',(0.,0.,-1.));
#64522=DIRECTION('center_axis',(1.,0.,0.));
#64523=DIRECTION('ref_axis',(0.,0.,-1.));
#64524=DIRECTION('',(1.,0.,0.));
#64525=DIRECTION('center_axis',(1.,0.,0.));
#64526=DIRECTION('ref_axis',(0.,0.,-1.));
#64527=DIRECTION('center_axis',(1.,0.,0.));
#64528=DIRECTION('ref_axis',(0.,0.,-1.));
#64529=DIRECTION('center_axis',(1.,0.,0.));
#64530=DIRECTION('ref_axis',(0.,0.,-1.));
#64531=DIRECTION('',(1.,0.,0.));
#64532=DIRECTION('center_axis',(1.,0.,0.));
#64533=DIRECTION('ref_axis',(0.,0.,-1.));
#64534=DIRECTION('center_axis',(1.,0.,0.));
#64535=DIRECTION('ref_axis',(0.,0.,-1.));
#64536=DIRECTION('center_axis',(1.,0.,0.));
#64537=DIRECTION('ref_axis',(0.,0.,-1.));
#64538=DIRECTION('',(1.,0.,0.));
#64539=DIRECTION('center_axis',(1.,0.,0.));
#64540=DIRECTION('ref_axis',(0.,0.,-1.));
#64541=DIRECTION('center_axis',(1.,0.,0.));
#64542=DIRECTION('ref_axis',(0.,0.,-1.));
#64543=DIRECTION('center_axis',(1.,0.,0.));
#64544=DIRECTION('ref_axis',(0.,0.,-1.));
#64545=DIRECTION('',(1.,0.,0.));
#64546=DIRECTION('center_axis',(1.,0.,0.));
#64547=DIRECTION('ref_axis',(0.,0.,-1.));
#64548=DIRECTION('center_axis',(1.,0.,0.));
#64549=DIRECTION('ref_axis',(0.,1.,0.));
#64550=DIRECTION('',(0.515038074910054,-0.857167300702112,-1.04972719113862E-16));
#64551=DIRECTION('center_axis',(1.,0.,0.));
#64552=DIRECTION('ref_axis',(0.,0.,-1.));
#64553=DIRECTION('center_axis',(1.,0.,0.));
#64554=DIRECTION('ref_axis',(0.,1.,0.));
#64555=DIRECTION('',(1.,0.,0.));
#64556=DIRECTION('center_axis',(1.,0.,0.));
#64557=DIRECTION('ref_axis',(0.,0.,-1.));
#64558=DIRECTION('center_axis',(1.,0.,0.));
#64559=DIRECTION('ref_axis',(0.,1.,0.));
#64560=DIRECTION('',(0.707106781186546,-0.707106781186549,-8.65956056235496E-17));
#64561=DIRECTION('center_axis',(-1.,0.,0.));
#64562=DIRECTION('ref_axis',(0.,1.,0.));
#64563=DIRECTION('center_axis',(1.,0.,0.));
#64564=DIRECTION('ref_axis',(0.,0.,-1.));
#64565=DIRECTION('center_axis',(0.,-1.,-1.22464679914735E-16));
#64566=DIRECTION('ref_axis',(0.,-1.22464679914735E-16,1.));
#64567=DIRECTION('center_axis',(-1.,0.,0.));
#64568=DIRECTION('ref_axis',(0.,-1.,1.83697019872103E-16));
#64569=DIRECTION('center_axis',(-1.,0.,0.));
#64570=DIRECTION('ref_axis',(0.,-1.,1.83697019872103E-16));
#64571=DIRECTION('center_axis',(1.,0.,0.));
#64572=DIRECTION('ref_axis',(0.,1.,0.));
#64573=DIRECTION('center_axis',(1.,0.,0.));
#64574=DIRECTION('ref_axis',(0.,0.,-1.));
#64575=DIRECTION('',(-1.,0.,0.));
#64576=DIRECTION('center_axis',(-1.,0.,0.));
#64577=DIRECTION('ref_axis',(0.,0.,1.));
#64578=DIRECTION('center_axis',(1.,0.,0.));
#64579=DIRECTION('ref_axis',(0.,0.,-1.));
#64580=DIRECTION('center_axis',(1.,0.,0.));
#64581=DIRECTION('ref_axis',(0.,1.,0.));
#64582=DIRECTION('center_axis',(1.,0.,0.));
#64583=DIRECTION('ref_axis',(0.,0.,-1.));
#64584=DIRECTION('',(-0.707106781186547,0.707106781186548,8.65956056235493E-17));
#64585=DIRECTION('center_axis',(1.,0.,0.));
#64586=DIRECTION('ref_axis',(0.,1.,0.));
#64587=DIRECTION('center_axis',(1.,0.,0.));
#64588=DIRECTION('ref_axis',(0.,0.,-1.));
#64589=DIRECTION('',(-1.,0.,0.));
#64590=DIRECTION('center_axis',(-1.,0.,0.));
#64591=DIRECTION('ref_axis',(0.,0.,1.));
#64592=DIRECTION('center_axis',(1.,0.,0.));
#64593=DIRECTION('ref_axis',(0.,0.,-1.));
#64594=DIRECTION('center_axis',(1.,0.,0.));
#64595=DIRECTION('ref_axis',(0.,1.,0.));
#64596=DIRECTION('center_axis',(1.,0.,0.));
#64597=DIRECTION('ref_axis',(0.,0.,-1.));
#64598=DIRECTION('',(-0.707106781186549,0.707106781186546,8.65956056235492E-17));
#64599=DIRECTION('center_axis',(1.,0.,0.));
#64600=DIRECTION('ref_axis',(0.,1.,0.));
#64601=DIRECTION('center_axis',(1.,0.,0.));
#64602=DIRECTION('ref_axis',(0.,0.,-1.));
#64603=DIRECTION('',(-1.,0.,0.));
#64604=DIRECTION('center_axis',(-1.,0.,0.));
#64605=DIRECTION('ref_axis',(0.,1.,0.));
#64606=DIRECTION('',(-0.707106781186548,-0.707106781186547,-8.65956056235492E-17));
#64607=DIRECTION('center_axis',(1.,0.,0.));
#64608=DIRECTION('ref_axis',(0.,0.,-1.));
#64609=DIRECTION('center_axis',(1.,0.,0.));
#64610=DIRECTION('ref_axis',(0.,0.,-1.));
#64611=DIRECTION('center_axis',(1.,0.,0.));
#64612=DIRECTION('ref_axis',(0.,1.,0.));
#64613=DIRECTION('center_axis',(1.,0.,0.));
#64614=DIRECTION('ref_axis',(0.,0.,-1.));
#64615=DIRECTION('',(-1.,0.,0.));
#64616=DIRECTION('center_axis',(-1.,0.,0.));
#64617=DIRECTION('ref_axis',(0.,1.,0.));
#64618=DIRECTION('center_axis',(1.,0.,0.));
#64619=DIRECTION('ref_axis',(0.,0.,-1.));
#64620=DIRECTION('',(-0.707106781186548,-0.707106781186547,-8.65956056235492E-17));
#64621=DIRECTION('center_axis',(1.,0.,0.));
#64622=DIRECTION('ref_axis',(0.,0.,-1.));
#80389=CARTESIAN_POINT('',(0.,0.,0.));
#80390=CARTESIAN_POINT('Origin',(11.85,-24.7487373415292,-24.7487373415292));
#80391=CARTESIAN_POINT('',(12.,-24.7487373415292,-21.4487373415292));
#80392=CARTESIAN_POINT('Origin',(12.,-24.7487373415292,-24.7487373415292));
#80393=CARTESIAN_POINT('',(11.7,-24.7487373415292,-21.7487373415292));
#80394=CARTESIAN_POINT('',(11.85,-24.7487373415292,-21.5987373415292));
#80395=CARTESIAN_POINT('Origin',(11.7,-24.7487373415292,-24.7487373415292));
#80396=CARTESIAN_POINT('Origin',(12.,20.,0.));
#80397=CARTESIAN_POINT('',(12.,-47.,-5.75583995599256E-15));
#80398=CARTESIAN_POINT('Origin',(12.,0.,0.));
#80399=CARTESIAN_POINT('',(12.,24.7487373415292,28.0487373415292));
#80400=CARTESIAN_POINT('Origin',(12.,24.7487373415292,24.7487373415292));
#80401=CARTESIAN_POINT('',(12.,-35.,5.50000000000001));
#80402=CARTESIAN_POINT('Origin',(12.,-35.,4.28626379701574E-15));
#80403=CARTESIAN_POINT('',(12.,2.81668763803891E-15,40.5));
#80404=CARTESIAN_POINT('Origin',(12.,2.14313189850787E-15,35.));
#80405=CARTESIAN_POINT('',(12.,35.,5.5));
#80406=CARTESIAN_POINT('Origin',(12.,35.,0.));
#80407=CARTESIAN_POINT('',(12.,-5.75583995599256E-15,-29.5));
#80408=CARTESIAN_POINT('Origin',(12.,-6.4293956955236E-15,-35.));
#80409=CARTESIAN_POINT('',(12.,-2.63299061816681E-15,21.5));
#80410=CARTESIAN_POINT('Origin',(12.,0.,0.));
#80411=CARTESIAN_POINT('Origin',(-0.5,-24.7487373415292,-24.7487373415292));
#80412=CARTESIAN_POINT('',(0.,-24.7487373415292,-21.7487373415292));
#80413=CARTESIAN_POINT('Origin',(0.,-24.7487373415292,-24.7487373415292));
#80414=CARTESIAN_POINT('',(-0.5,-24.7487373415292,-21.7487373415292));
#80415=CARTESIAN_POINT('Origin',(11.85,24.7487373415292,24.7487373415292));
#80416=CARTESIAN_POINT('',(11.7,24.7487373415292,27.7487373415292));
#80417=CARTESIAN_POINT('',(11.85,24.7487373415292,27.8987373415292));
#80418=CARTESIAN_POINT('Origin',(11.7,24.7487373415292,24.7487373415292));
#80419=CARTESIAN_POINT('Origin',(-0.5,24.7487373415292,24.7487373415292));
#80420=CARTESIAN_POINT('',(0.,24.7487373415292,27.7487373415292));
#80421=CARTESIAN_POINT('Origin',(0.,24.7487373415292,24.7487373415292));
#80422=CARTESIAN_POINT('',(-0.5,24.7487373415292,27.7487373415292));
#80423=CARTESIAN_POINT('Origin',(-0.5,35.,0.));
#80424=CARTESIAN_POINT('',(0.,35.,3.3));
#80425=CARTESIAN_POINT('Origin',(0.,35.,0.));
#80426=CARTESIAN_POINT('',(5.5,35.,3.3));
#80427=CARTESIAN_POINT('',(-0.5,35.,3.3));
#80428=CARTESIAN_POINT('Origin',(5.5,35.,0.));
#80429=CARTESIAN_POINT('Origin',(-0.5,2.14313189850787E-15,35.));
#80430=CARTESIAN_POINT('',(0.,1.73899845478924E-15,38.3));
#80431=CARTESIAN_POINT('Origin',(0.,2.14313189850787E-15,35.));
#80432=CARTESIAN_POINT('',(5.5,2.54726534222649E-15,38.3));
#80433=CARTESIAN_POINT('',(-0.5,1.73899845478924E-15,38.3));
#80434=CARTESIAN_POINT('Origin',(5.5,2.14313189850787E-15,35.));
#80435=CARTESIAN_POINT('Origin',(-0.5,-35.,4.28626379701574E-15));
#80436=CARTESIAN_POINT('',(0.,-35.,3.3));
#80437=CARTESIAN_POINT('Origin',(0.,-35.,4.28626379701574E-15));
#80438=CARTESIAN_POINT('',(5.5,-35.,3.3));
#80439=CARTESIAN_POINT('',(-0.5,-35.,3.3));
#80440=CARTESIAN_POINT('Origin',(5.5,-35.,4.28626379701574E-15));
#80441=CARTESIAN_POINT('Origin',(-0.5,-6.4293956955236E-15,-35.));
#80442=CARTESIAN_POINT('',(0.,-6.83352913924223E-15,-31.7));
#80443=CARTESIAN_POINT('Origin',(0.,-6.4293956955236E-15,-35.));
#80444=CARTESIAN_POINT('',(5.5,-6.02526225180498E-15,-31.7));
#80445=CARTESIAN_POINT('',(-0.5,-6.83352913924223E-15,-31.7));
#80446=CARTESIAN_POINT('Origin',(5.5,-6.4293956955236E-15,-35.));
#80447=CARTESIAN_POINT('Origin',(5.5,-35.,4.28626379701574E-15));
#80448=CARTESIAN_POINT('',(5.5,-35.,5.50000000000001));
#80449=CARTESIAN_POINT('Origin',(5.5,-35.,4.28626379701574E-15));
#80450=CARTESIAN_POINT('',(5.5,-35.,5.50000000000001));
#80451=CARTESIAN_POINT('Origin',(5.5,-35.,4.44089209850063E-15));
#80452=CARTESIAN_POINT('Origin',(5.5,2.14313189850787E-15,35.));
#80453=CARTESIAN_POINT('',(5.5,1.46957615897682E-15,40.5));
#80454=CARTESIAN_POINT('Origin',(5.5,2.14313189850787E-15,35.));
#80455=CARTESIAN_POINT('',(5.5,1.46957615897682E-15,40.5));
#80456=CARTESIAN_POINT('Origin',(5.5,2.22044604925031E-15,35.));
#80457=CARTESIAN_POINT('Origin',(5.5,35.,0.));
#80458=CARTESIAN_POINT('',(5.5,35.,5.5));
#80459=CARTESIAN_POINT('Origin',(5.5,35.,0.));
#80460=CARTESIAN_POINT('',(5.5,35.,5.5));
#80461=CARTESIAN_POINT('Origin',(5.5,35.,0.));
#80462=CARTESIAN_POINT('Origin',(5.5,-6.4293956955236E-15,-35.));
#80463=CARTESIAN_POINT('',(5.5,-7.10295143505465E-15,-29.5));
#80464=CARTESIAN_POINT('Origin',(5.5,-6.4293956955236E-15,-35.));
#80465=CARTESIAN_POINT('',(5.5,-7.10295143505465E-15,-29.5));
#80466=CARTESIAN_POINT('Origin',(5.5,-6.66133814775094E-15,-35.));
#80467=CARTESIAN_POINT('Origin',(18.4828269369554,0.,0.));
#80468=CARTESIAN_POINT('',(16.9656538739108,0.,0.));
#80469=CARTESIAN_POINT('',(20.,-5.05,-6.18446633569413E-16));
#80470=CARTESIAN_POINT('',(18.4828269369554,-2.525,-3.09223316784707E-16));
#80471=CARTESIAN_POINT('Origin',(20.,0.,0.));
#80472=CARTESIAN_POINT('Origin',(29.75,0.,0.));
#80473=CARTESIAN_POINT('',(39.5,-5.05,-6.18446633569413E-16));
#80474=CARTESIAN_POINT('',(29.75,-5.05,-6.18446633569413E-16));
#80475=CARTESIAN_POINT('Origin',(39.5,0.,0.));
#80476=CARTESIAN_POINT('Origin',(39.8,0.,0.));
#80477=CARTESIAN_POINT('',(40.,-5.55,6.79678973526781E-16));
#80478=CARTESIAN_POINT('',(39.8,-5.35,-6.55186037543834E-16));
#80479=CARTESIAN_POINT('Origin',(40.,0.,0.));
#80480=CARTESIAN_POINT('Origin',(13.5,0.,0.));
#80481=CARTESIAN_POINT('',(13.5,-2.44929359829471E-15,20.));
#80482=CARTESIAN_POINT('Origin',(13.5,-2.63299061816681E-15,21.5));
#80483=CARTESIAN_POINT('',(13.5,-20.,-2.44929359829471E-15));
#80484=CARTESIAN_POINT('Origin',(13.5,0.,0.));
#80485=CARTESIAN_POINT('Origin',(13.5,0.,0.));
#80486=CARTESIAN_POINT('Origin',(15.25,0.,0.));
#80487=CARTESIAN_POINT('',(18.5,-20.,-2.44929359829471E-15));
#80488=CARTESIAN_POINT('Origin',(18.5,0.,0.));
#80489=CARTESIAN_POINT('',(15.25,-20.,-2.44929359829471E-15));
#80490=CARTESIAN_POINT('Origin',(-4.,19.5,0.));
#80491=CARTESIAN_POINT('',(-4.,-19.5,-2.38806125833734E-15));
#80492=CARTESIAN_POINT('Origin',(-4.,0.,0.));
#80493=CARTESIAN_POINT('Origin',(-3.75,0.,0.));
#80494=CARTESIAN_POINT('',(-3.5,-20.,-2.44929359829471E-15));
#80495=CARTESIAN_POINT('Origin',(-3.5,0.,0.));
#80496=CARTESIAN_POINT('',(-3.75,-19.75,-2.41867742831602E-15));
#80497=CARTESIAN_POINT('Origin',(-1.75,0.,0.));
#80498=CARTESIAN_POINT('',(0.,-20.,-2.44929359829471E-15));
#80499=CARTESIAN_POINT('Origin',(0.,0.,0.));
#80500=CARTESIAN_POINT('',(-1.75,-20.,-2.44929359829471E-15));
#80501=CARTESIAN_POINT('Origin',(0.,47.,0.));
#80502=CARTESIAN_POINT('',(-2.35922392732846E-15,-47.,-5.75583995599256E-15));
#80503=CARTESIAN_POINT('Origin',(0.,0.,0.));
#80504=CARTESIAN_POINT('Origin',(0.499999999999998,0.,0.));
#80505=CARTESIAN_POINT('',(1.,-48.,-5.8783046359073E-15));
#80506=CARTESIAN_POINT('Origin',(1.,0.,0.));
#80507=CARTESIAN_POINT('',(0.499999999999998,-47.5,-5.81707229594993E-15));
#80508=CARTESIAN_POINT('Origin',(6.,0.,0.));
#80509=CARTESIAN_POINT('',(11.,-48.,-5.8783046359073E-15));
#80510=CARTESIAN_POINT('Origin',(11.,0.,0.));
#80511=CARTESIAN_POINT('',(6.,-48.,-5.8783046359073E-15));
#80512=CARTESIAN_POINT('Origin',(11.5,0.,0.));
#80513=CARTESIAN_POINT('',(11.5,-47.5,-5.81707229594993E-15));
#80514=CARTESIAN_POINT('Origin',(18.5,14.995,0.));
#80515=CARTESIAN_POINT('',(18.5,-14.995,-1.83635787532146E-15));
#80516=CARTESIAN_POINT('Origin',(18.5,0.,0.));
#80517=CARTESIAN_POINT('Origin',(28.75,0.,0.));
#80518=CARTESIAN_POINT('',(39.,-14.995,-1.83635787532146E-15));
#80519=CARTESIAN_POINT('Origin',(39.,0.,0.));
#80520=CARTESIAN_POINT('',(28.75,-14.995,-1.83635787532146E-15));
#80521=CARTESIAN_POINT('Origin',(39.5,0.,0.));
#80522=CARTESIAN_POINT('',(40.,-13.995,-1.71389319540672E-15));
#80523=CARTESIAN_POINT('Origin',(40.,0.,0.));
#80524=CARTESIAN_POINT('',(39.5,-14.495,-1.77512553536409E-15));
#80525=CARTESIAN_POINT('Origin',(40.,0.,0.));
#94273=UNCERTAINTY_MEASURE_WITH_UNIT(LENGTH_MEASURE(0.01),#94302,
'DISTANCE_ACCURACY_VALUE',
'Maximum model space distance between geometric entities at asserted c
onnectivities');
#94285=UNCERTAINTY_MEASURE_WITH_UNIT(LENGTH_MEASURE(0.01),#94302,
'DISTANCE_ACCURACY_VALUE',
'Maximum model space distance between geometric entities at asserted c
onnectivities');
#94289=(
GEOMETRIC_REPRESENTATION_CONTEXT(3)
GLOBAL_UNCERTAINTY_ASSIGNED_CONTEXT((#94273))
GLOBAL_UNIT_ASSIGNED_CONTEXT((#94302,#94304,#94305))
REPRESENTATION_CONTEXT('','3D')
);
#94301=(
GEOMETRIC_REPRESENTATION_CONTEXT(3)
GLOBAL_UNCERTAINTY_ASSIGNED_CONTEXT((#94285))
GLOBAL_UNIT_ASSIGNED_CONTEXT((#94302,#94304,#94305))
REPRESENTATION_CONTEXT('','3D')
);
#94302=(
LENGTH_UNIT()
NAMED_UNIT(*)
SI_UNIT(.MILLI.,.METRE.)
);
#94304=(
NAMED_UNIT(*)
PLANE_ANGLE_UNIT()
SI_UNIT($,.RADIAN.)
);
#94305=(
NAMED_UNIT(*)
SI_UNIT($,.STERADIAN.)
SOLID_ANGLE_UNIT()
);
#94309=SHAPE_DEFINITION_REPRESENTATION(#94324,#94373);
#94324=PRODUCT_DEFINITION_SHAPE('',$,#94389);
#94373=SHAPE_REPRESENTATION('',(#54142),#94289);
#94385=PRODUCT_DEFINITION_CONTEXT('part definition',#94432,'design');
#94389=PRODUCT_DEFINITION('2026-10-11-08-26-34-261',
'03_Display_Pedestal',#94404,#94385);
#94404=PRODUCT_DEFINITION_FORMATION('',$,#94437);
#94432=APPLICATION_CONTEXT(
'Core Data for Automotive Mechanical Design Process');
#94433=PRODUCT_CONTEXT('part definition',#94432,'mechanical');
#94437=PRODUCT('2026-10-11-08-26-34-261','03_Display_Pedestal',$,(#94433));
#94568=COLOUR_RGB('Sky Blue',0.24,0.69,0.87);
#94569=FILL_AREA_STYLE_COLOUR('',#94568);
#94570=FILL_AREA_STYLE('',(#94569));
#94571=SURFACE_STYLE_FILL_AREA(#94570);
#94572=SURFACE_SIDE_STYLE('',(#94571));
#94573=SURFACE_STYLE_USAGE(.BOTH.,#94572);
#94574=PRESENTATION_STYLE_ASSIGNMENT((#94573));
ENDSEC;
END-ISO-10303-21;
